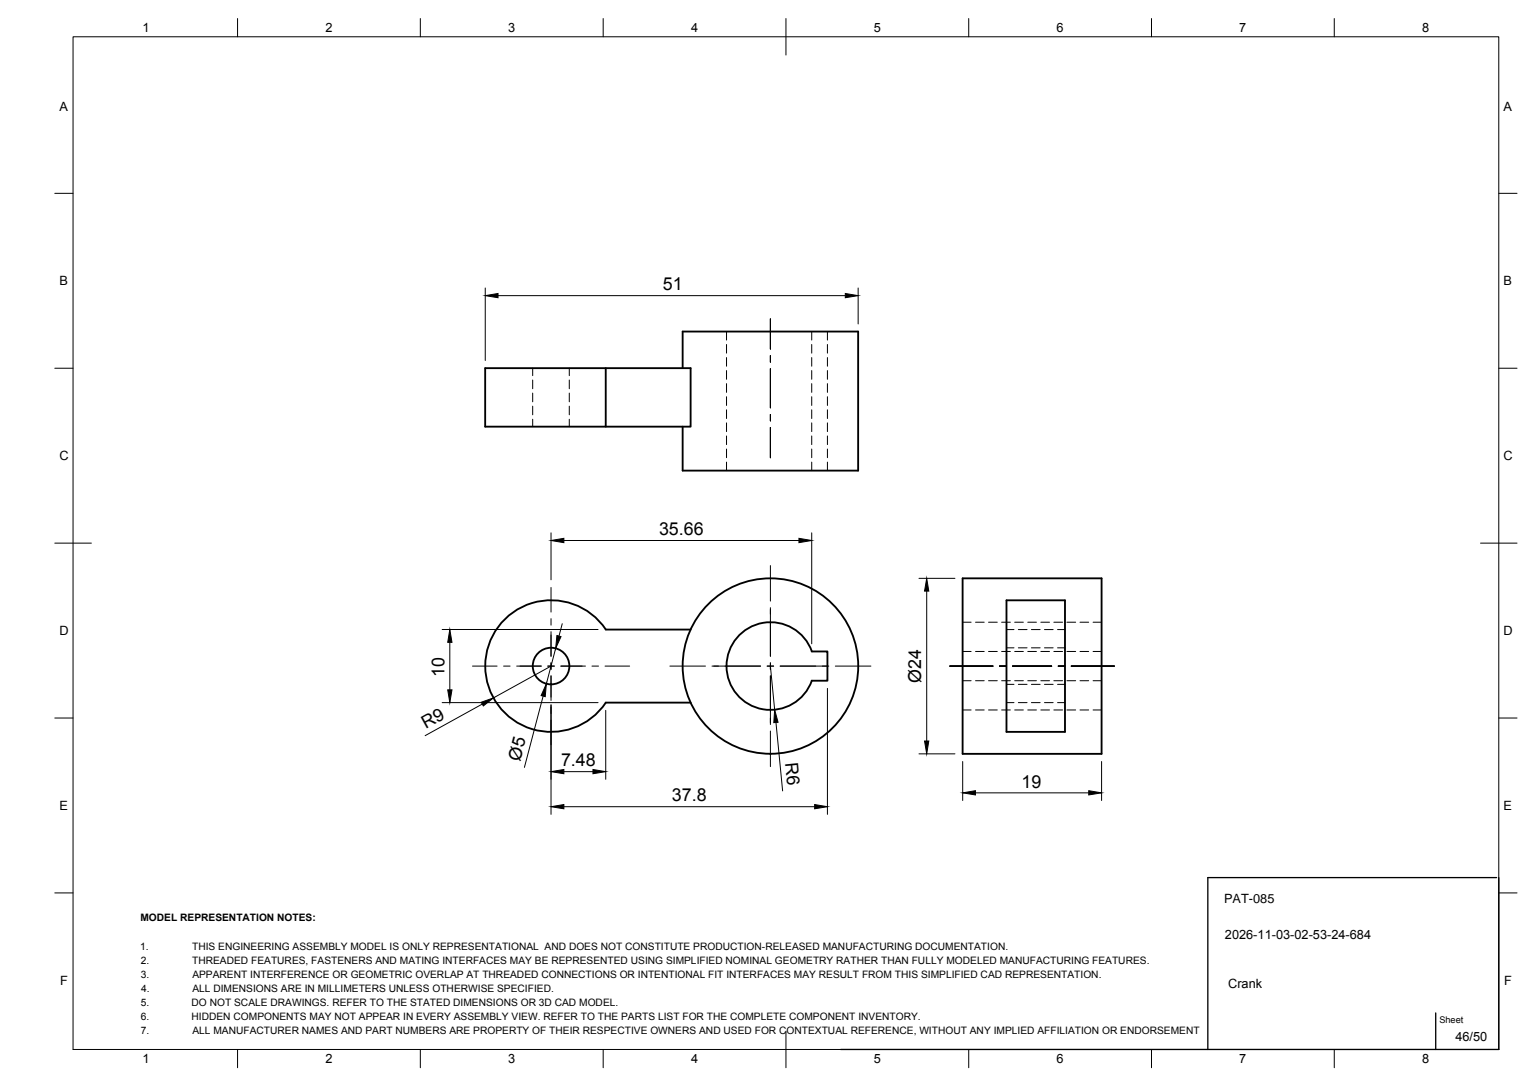
ISO-10303-21;
HEADER;
/* Generated by software containing ST-Developer
 * from STEP Tools, Inc. (www.steptools.com) 
 */

FILE_DESCRIPTION(
/* description */ ('Rack and pinion manual slide'),
/* implementation_level */ '2;1');

FILE_NAME(
/* name */ 'Crank.step',
/* time_stamp */ '2026-10-28T03:22:49-07:00',
/* author */ (''),
/* organization */ (''),
/* preprocessor_version */ 'ST-DEVELOPER v20.2',
/* originating_system */ 'Autodesk Translation Framework v15.17.0.0',
/* authorisation */ '');

FILE_SCHEMA (('AUTOMOTIVE_DESIGN { 1 0 10303 214 3 1 1 }'));
ENDSEC;

DATA;
#10=MECHANICAL_DESIGN_GEOMETRIC_PRESENTATION_REPRESENTATION('',(#777),#34851);
#678=SHAPE_REPRESENTATION_RELATIONSHIP('SRR','None',#35117,#724);
#724=ADVANCED_BREP_SHAPE_REPRESENTATION('',(#827),#34842);
#777=STYLED_ITEM('',(#35425),#827);
#827=MANIFOLD_SOLID_BREP('Body1',#13800);
#1028=FACE_BOUND('',#3056,.T.);
#1029=FACE_BOUND('',#3061,.T.);
#1030=FACE_BOUND('',#3064,.T.);
#1031=FACE_BOUND('',#3066,.T.);
#1032=FACE_BOUND('',#3068,.T.);
#1462=PLANE('',#15293);
#1463=PLANE('',#15294);
#1464=PLANE('',#15295);
#1465=PLANE('',#15296);
#1466=PLANE('',#15304);
#1467=PLANE('',#15305);
#1468=PLANE('',#15307);
#1469=PLANE('',#15308);
#1470=PLANE('',#15312);
#2117=FACE_OUTER_BOUND('',#3051,.T.);
#2118=FACE_OUTER_BOUND('',#3052,.T.);
#2119=FACE_OUTER_BOUND('',#3053,.T.);
#2120=FACE_OUTER_BOUND('',#3054,.T.);
#2121=FACE_OUTER_BOUND('',#3055,.T.);
#2122=FACE_OUTER_BOUND('',#3057,.T.);
#2123=FACE_OUTER_BOUND('',#3058,.T.);
#2124=FACE_OUTER_BOUND('',#3059,.T.);
#2125=FACE_OUTER_BOUND('',#3060,.T.);
#2126=FACE_OUTER_BOUND('',#3062,.T.);
#2127=FACE_OUTER_BOUND('',#3063,.T.);
#2128=FACE_OUTER_BOUND('',#3065,.T.);
#2129=FACE_OUTER_BOUND('',#3067,.T.);
#3051=EDGE_LOOP('',(#12062,#12063,#12064,#12065));
#3052=EDGE_LOOP('',(#12066,#12067,#12068,#12069));
#3053=EDGE_LOOP('',(#12070,#12071,#12072,#12073));
#3054=EDGE_LOOP('',(#12074,#12075,#12076,#12077));
#3055=EDGE_LOOP('',(#12078));
#3056=EDGE_LOOP('',(#12079,#12080,#12081,#12082));
#3057=EDGE_LOOP('',(#12083,#12084,#12085,#12086));
#3058=EDGE_LOOP('',(#12087,#12088,#12089,#12090));
#3059=EDGE_LOOP('',(#12091,#12092,#12093,#12094));
#3060=EDGE_LOOP('',(#12095,#12096,#12097,#12098));
#3061=EDGE_LOOP('',(#12099));
#3062=EDGE_LOOP('',(#12100,#12101,#12102,#12103));
#3063=EDGE_LOOP('',(#12104,#12105,#12106,#12107));
#3064=EDGE_LOOP('',(#12108));
#3065=EDGE_LOOP('',(#12109,#12110,#12111,#12112));
#3066=EDGE_LOOP('',(#12113,#12114,#12115,#12116));
#3067=EDGE_LOOP('',(#12117));
#3068=EDGE_LOOP('',(#12118,#12119,#12120,#12121));
#4286=LINE('',#22751,#5577);
#4287=LINE('',#22756,#5578);
#4288=LINE('',#22758,#5579);
#4289=LINE('',#22760,#5580);
#4290=LINE('',#22761,#5581);
#4291=LINE('',#22764,#5582);
#4292=LINE('',#22766,#5583);
#4293=LINE('',#22767,#5584);
#4294=LINE('',#22770,#5585);
#4295=LINE('',#22772,#5586);
#4296=LINE('',#22773,#5587);
#4297=LINE('',#22783,#5588);
#4298=LINE('',#22787,#5589);
#4299=LINE('',#22791,#5590);
#4300=LINE('',#22793,#5591);
#4301=LINE('',#22794,#5592);
#4302=LINE('',#22797,#5593);
#4303=LINE('',#22801,#5594);
#4304=LINE('',#22802,#5595);
#4305=LINE('',#22807,#5596);
#5577=VECTOR('',#18612,0.25);
#5578=VECTOR('',#18617,1.);
#5579=VECTOR('',#18618,1.);
#5580=VECTOR('',#18619,1.);
#5581=VECTOR('',#18620,1.);
#5582=VECTOR('',#18623,1.);
#5583=VECTOR('',#18624,1.);
#5584=VECTOR('',#18625,1.);
#5585=VECTOR('',#18628,1.);
#5586=VECTOR('',#18629,1.);
#5587=VECTOR('',#18630,1.);
#5588=VECTOR('',#18643,1.);
#5589=VECTOR('',#18646,1.);
#5590=VECTOR('',#18651,1.);
#5591=VECTOR('',#18652,1.);
#5592=VECTOR('',#18653,1.);
#5593=VECTOR('',#18656,1.);
#5594=VECTOR('',#18661,1.);
#5595=VECTOR('',#18662,1.);
#5596=VECTOR('',#18669,1.2);
#6142=CIRCLE('',#15291,0.25);
#6143=CIRCLE('',#15292,0.25);
#6144=CIRCLE('',#15297,1.2);
#6145=CIRCLE('',#15298,0.6);
#6146=CIRCLE('',#15300,0.6);
#6147=CIRCLE('',#15302,0.9);
#6148=CIRCLE('',#15303,0.9);
#6149=CIRCLE('',#15306,1.2);
#6150=CIRCLE('',#15309,1.2);
#6151=CIRCLE('',#15311,1.2);
#7171=VERTEX_POINT('',#22748);
#7172=VERTEX_POINT('',#22750);
#7173=VERTEX_POINT('',#22754);
#7174=VERTEX_POINT('',#22755);
#7175=VERTEX_POINT('',#22757);
#7176=VERTEX_POINT('',#22759);
#7177=VERTEX_POINT('',#22763);
#7178=VERTEX_POINT('',#22765);
#7179=VERTEX_POINT('',#22769);
#7180=VERTEX_POINT('',#22771);
#7181=VERTEX_POINT('',#22775);
#7182=VERTEX_POINT('',#22781);
#7183=VERTEX_POINT('',#22782);
#7184=VERTEX_POINT('',#22784);
#7185=VERTEX_POINT('',#22786);
#7186=VERTEX_POINT('',#22790);
#7187=VERTEX_POINT('',#22792);
#7188=VERTEX_POINT('',#22796);
#7189=VERTEX_POINT('',#22800);
#7190=VERTEX_POINT('',#22806);
#8843=EDGE_CURVE('',#7171,#7171,#6142,.T.);
#8844=EDGE_CURVE('',#7171,#7172,#4286,.T.);
#8845=EDGE_CURVE('',#7172,#7172,#6143,.T.);
#8846=EDGE_CURVE('',#7173,#7174,#4287,.T.);
#8847=EDGE_CURVE('',#7173,#7175,#4288,.T.);
#8848=EDGE_CURVE('',#7176,#7175,#4289,.T.);
#8849=EDGE_CURVE('',#7174,#7176,#4290,.T.);
#8850=EDGE_CURVE('',#7177,#7173,#4291,.T.);
#8851=EDGE_CURVE('',#7177,#7178,#4292,.T.);
#8852=EDGE_CURVE('',#7175,#7178,#4293,.T.);
#8853=EDGE_CURVE('',#7179,#7177,#4294,.T.);
#8854=EDGE_CURVE('',#7180,#7179,#4295,.T.);
#8855=EDGE_CURVE('',#7178,#7180,#4296,.T.);
#8856=EDGE_CURVE('',#7181,#7181,#6144,.T.);
#8857=EDGE_CURVE('',#7180,#7176,#6145,.T.);
#8858=EDGE_CURVE('',#7179,#7174,#6146,.T.);
#8859=EDGE_CURVE('',#7182,#7183,#4297,.T.);
#8860=EDGE_CURVE('',#7184,#7182,#6147,.T.);
#8861=EDGE_CURVE('',#7185,#7184,#4298,.T.);
#8862=EDGE_CURVE('',#7185,#7183,#6148,.T.);
#8863=EDGE_CURVE('',#7186,#7183,#4299,.T.);
#8864=EDGE_CURVE('',#7187,#7186,#4300,.T.);
#8865=EDGE_CURVE('',#7182,#7187,#4301,.T.);
#8866=EDGE_CURVE('',#7185,#7188,#4302,.T.);
#8867=EDGE_CURVE('',#7186,#7188,#6149,.T.);
#8868=EDGE_CURVE('',#7189,#7184,#4303,.T.);
#8869=EDGE_CURVE('',#7188,#7189,#4304,.T.);
#8870=EDGE_CURVE('',#7189,#7187,#6150,.T.);
#8871=EDGE_CURVE('',#7181,#7190,#4305,.T.);
#8872=EDGE_CURVE('',#7190,#7190,#6151,.T.);
#12062=ORIENTED_EDGE('',*,*,#8843,.F.);
#12063=ORIENTED_EDGE('',*,*,#8844,.T.);
#12064=ORIENTED_EDGE('',*,*,#8845,.F.);
#12065=ORIENTED_EDGE('',*,*,#8844,.F.);
#12066=ORIENTED_EDGE('',*,*,#8846,.F.);
#12067=ORIENTED_EDGE('',*,*,#8847,.T.);
#12068=ORIENTED_EDGE('',*,*,#8848,.F.);
#12069=ORIENTED_EDGE('',*,*,#8849,.F.);
#12070=ORIENTED_EDGE('',*,*,#8850,.F.);
#12071=ORIENTED_EDGE('',*,*,#8851,.T.);
#12072=ORIENTED_EDGE('',*,*,#8852,.F.);
#12073=ORIENTED_EDGE('',*,*,#8847,.F.);
#12074=ORIENTED_EDGE('',*,*,#8853,.F.);
#12075=ORIENTED_EDGE('',*,*,#8854,.F.);
#12076=ORIENTED_EDGE('',*,*,#8855,.F.);
#12077=ORIENTED_EDGE('',*,*,#8851,.F.);
#12078=ORIENTED_EDGE('',*,*,#8856,.T.);
#12079=ORIENTED_EDGE('',*,*,#8848,.T.);
#12080=ORIENTED_EDGE('',*,*,#8852,.T.);
#12081=ORIENTED_EDGE('',*,*,#8855,.T.);
#12082=ORIENTED_EDGE('',*,*,#8857,.T.);
#12083=ORIENTED_EDGE('',*,*,#8849,.T.);
#12084=ORIENTED_EDGE('',*,*,#8857,.F.);
#12085=ORIENTED_EDGE('',*,*,#8854,.T.);
#12086=ORIENTED_EDGE('',*,*,#8858,.T.);
#12087=ORIENTED_EDGE('',*,*,#8859,.F.);
#12088=ORIENTED_EDGE('',*,*,#8860,.F.);
#12089=ORIENTED_EDGE('',*,*,#8861,.F.);
#12090=ORIENTED_EDGE('',*,*,#8862,.T.);
#12091=ORIENTED_EDGE('',*,*,#8859,.T.);
#12092=ORIENTED_EDGE('',*,*,#8863,.F.);
#12093=ORIENTED_EDGE('',*,*,#8864,.F.);
#12094=ORIENTED_EDGE('',*,*,#8865,.F.);
#12095=ORIENTED_EDGE('',*,*,#8862,.F.);
#12096=ORIENTED_EDGE('',*,*,#8866,.T.);
#12097=ORIENTED_EDGE('',*,*,#8867,.F.);
#12098=ORIENTED_EDGE('',*,*,#8863,.T.);
#12099=ORIENTED_EDGE('',*,*,#8843,.T.);
#12100=ORIENTED_EDGE('',*,*,#8861,.T.);
#12101=ORIENTED_EDGE('',*,*,#8868,.F.);
#12102=ORIENTED_EDGE('',*,*,#8869,.F.);
#12103=ORIENTED_EDGE('',*,*,#8866,.F.);
#12104=ORIENTED_EDGE('',*,*,#8865,.T.);
#12105=ORIENTED_EDGE('',*,*,#8870,.F.);
#12106=ORIENTED_EDGE('',*,*,#8868,.T.);
#12107=ORIENTED_EDGE('',*,*,#8860,.T.);
#12108=ORIENTED_EDGE('',*,*,#8845,.T.);
#12109=ORIENTED_EDGE('',*,*,#8856,.F.);
#12110=ORIENTED_EDGE('',*,*,#8871,.T.);
#12111=ORIENTED_EDGE('',*,*,#8872,.T.);
#12112=ORIENTED_EDGE('',*,*,#8871,.F.);
#12113=ORIENTED_EDGE('',*,*,#8864,.T.);
#12114=ORIENTED_EDGE('',*,*,#8867,.T.);
#12115=ORIENTED_EDGE('',*,*,#8869,.T.);
#12116=ORIENTED_EDGE('',*,*,#8870,.T.);
#12117=ORIENTED_EDGE('',*,*,#8872,.F.);
#12118=ORIENTED_EDGE('',*,*,#8846,.T.);
#12119=ORIENTED_EDGE('',*,*,#8858,.F.);
#12120=ORIENTED_EDGE('',*,*,#8853,.T.);
#12121=ORIENTED_EDGE('',*,*,#8850,.T.);
#12977=CYLINDRICAL_SURFACE('',#15290,0.25);
#12978=CYLINDRICAL_SURFACE('',#15299,0.6);
#12979=CYLINDRICAL_SURFACE('',#15301,0.9);
#12980=CYLINDRICAL_SURFACE('',#15310,1.2);
#13595=ADVANCED_FACE('',(#2117),#12977,.F.);
#13596=ADVANCED_FACE('',(#2118),#1462,.F.);
#13597=ADVANCED_FACE('',(#2119),#1463,.F.);
#13598=ADVANCED_FACE('',(#2120),#1464,.F.);
#13599=ADVANCED_FACE('',(#2121,#1028),#1465,.T.);
#13600=ADVANCED_FACE('',(#2122),#12978,.F.);
#13601=ADVANCED_FACE('',(#2123),#12979,.T.);
#13602=ADVANCED_FACE('',(#2124),#1466,.T.);
#13603=ADVANCED_FACE('',(#2125,#1029),#1467,.F.);
#13604=ADVANCED_FACE('',(#2126),#1468,.T.);
#13605=ADVANCED_FACE('',(#2127,#1030),#1469,.T.);
#13606=ADVANCED_FACE('',(#2128,#1031),#12980,.T.);
#13607=ADVANCED_FACE('',(#2129,#1032),#1470,.F.);
#13800=CLOSED_SHELL('',(#13595,#13596,#13597,#13598,#13599,#13600,#13601,
#13602,#13603,#13604,#13605,#13606,#13607));
#15289=AXIS2_PLACEMENT_3D('',#22746,#18606,#18607);
#15290=AXIS2_PLACEMENT_3D('',#22747,#18608,#18609);
#15291=AXIS2_PLACEMENT_3D('',#22749,#18610,#18611);
#15292=AXIS2_PLACEMENT_3D('',#22752,#18613,#18614);
#15293=AXIS2_PLACEMENT_3D('',#22753,#18615,#18616);
#15294=AXIS2_PLACEMENT_3D('',#22762,#18621,#18622);
#15295=AXIS2_PLACEMENT_3D('',#22768,#18626,#18627);
#15296=AXIS2_PLACEMENT_3D('',#22774,#18631,#18632);
#15297=AXIS2_PLACEMENT_3D('',#22776,#18633,#18634);
#15298=AXIS2_PLACEMENT_3D('',#22777,#18635,#18636);
#15299=AXIS2_PLACEMENT_3D('',#22778,#18637,#18638);
#15300=AXIS2_PLACEMENT_3D('',#22779,#18639,#18640);
#15301=AXIS2_PLACEMENT_3D('',#22780,#18641,#18642);
#15302=AXIS2_PLACEMENT_3D('',#22785,#18644,#18645);
#15303=AXIS2_PLACEMENT_3D('',#22788,#18647,#18648);
#15304=AXIS2_PLACEMENT_3D('',#22789,#18649,#18650);
#15305=AXIS2_PLACEMENT_3D('',#22795,#18654,#18655);
#15306=AXIS2_PLACEMENT_3D('',#22798,#18657,#18658);
#15307=AXIS2_PLACEMENT_3D('',#22799,#18659,#18660);
#15308=AXIS2_PLACEMENT_3D('',#22803,#18663,#18664);
#15309=AXIS2_PLACEMENT_3D('',#22804,#18665,#18666);
#15310=AXIS2_PLACEMENT_3D('',#22805,#18667,#18668);
#15311=AXIS2_PLACEMENT_3D('',#22808,#18670,#18671);
#15312=AXIS2_PLACEMENT_3D('',#22809,#18672,#18673);
#18606=DIRECTION('axis',(0.,0.,1.));
#18607=DIRECTION('refdir',(1.,0.,0.));
#18608=DIRECTION('center_axis',(0.,1.,0.));
#18609=DIRECTION('ref_axis',(1.,0.,0.));
#18610=DIRECTION('center_axis',(0.,1.,0.));
#18611=DIRECTION('ref_axis',(1.,0.,0.));
#18612=DIRECTION('',(0.,1.,0.));
#18613=DIRECTION('center_axis',(0.,-1.,0.));
#18614=DIRECTION('ref_axis',(1.,0.,0.));
#18615=DIRECTION('center_axis',(-1.,0.,0.));
#18616=DIRECTION('ref_axis',(0.,0.,1.));
#18617=DIRECTION('',(0.,0.,1.));
#18618=DIRECTION('',(0.,1.,0.));
#18619=DIRECTION('',(0.,0.,-1.));
#18620=DIRECTION('',(0.,1.,0.));
#18621=DIRECTION('center_axis',(0.,0.,-1.));
#18622=DIRECTION('ref_axis',(-1.,0.,0.));
#18623=DIRECTION('',(-1.,0.,0.));
#18624=DIRECTION('',(0.,1.,0.));
#18625=DIRECTION('',(1.,0.,0.));
#18626=DIRECTION('center_axis',(1.,0.,0.));
#18627=DIRECTION('ref_axis',(0.,0.,-1.));
#18628=DIRECTION('',(0.,0.,-1.));
#18629=DIRECTION('',(0.,-1.,0.));
#18630=DIRECTION('',(0.,0.,1.));
#18631=DIRECTION('center_axis',(0.,1.,0.));
#18632=DIRECTION('ref_axis',(1.,0.,0.));
#18633=DIRECTION('center_axis',(0.,1.,0.));
#18634=DIRECTION('ref_axis',(1.,0.,0.));
#18635=DIRECTION('center_axis',(0.,-1.,0.));
#18636=DIRECTION('ref_axis',(1.,0.,0.));
#18637=DIRECTION('center_axis',(0.,1.,0.));
#18638=DIRECTION('ref_axis',(-1.83697019872103E-16,0.,1.));
#18639=DIRECTION('center_axis',(0.,-1.,0.));
#18640=DIRECTION('ref_axis',(1.,0.,0.));
#18641=DIRECTION('center_axis',(0.,1.,0.));
#18642=DIRECTION('ref_axis',(6.12323399573677E-17,0.,1.));
#18643=DIRECTION('',(0.,-1.,0.));
#18644=DIRECTION('center_axis',(0.,1.,0.));
#18645=DIRECTION('ref_axis',(1.,0.,0.));
#18646=DIRECTION('',(0.,1.,0.));
#18647=DIRECTION('center_axis',(0.,1.,0.));
#18648=DIRECTION('ref_axis',(1.,0.,0.));
#18649=DIRECTION('center_axis',(1.,0.,0.));
#18650=DIRECTION('ref_axis',(0.,0.,-1.));
#18651=DIRECTION('',(0.,0.,1.));
#18652=DIRECTION('',(0.,-1.,0.));
#18653=DIRECTION('',(0.,0.,-1.));
#18654=DIRECTION('center_axis',(0.,1.,0.));
#18655=DIRECTION('ref_axis',(1.,0.,0.));
#18656=DIRECTION('',(0.,0.,-1.));
#18657=DIRECTION('center_axis',(0.,-1.,0.));
#18658=DIRECTION('ref_axis',(1.,0.,0.));
#18659=DIRECTION('center_axis',(-1.,0.,0.));
#18660=DIRECTION('ref_axis',(0.,0.,1.));
#18661=DIRECTION('',(0.,0.,1.));
#18662=DIRECTION('',(0.,1.,0.));
#18663=DIRECTION('center_axis',(0.,1.,0.));
#18664=DIRECTION('ref_axis',(0.,0.,1.));
#18665=DIRECTION('center_axis',(0.,1.,0.));
#18666=DIRECTION('ref_axis',(1.,0.,0.));
#18667=DIRECTION('center_axis',(0.,1.,0.));
#18668=DIRECTION('ref_axis',(1.,0.,0.));
#18669=DIRECTION('',(0.,-1.,0.));
#18670=DIRECTION('center_axis',(0.,1.,0.));
#18671=DIRECTION('ref_axis',(1.,0.,0.));
#18672=DIRECTION('center_axis',(0.,1.,0.));
#18673=DIRECTION('ref_axis',(1.,0.,0.));
#22746=CARTESIAN_POINT('',(0.,0.,0.));
#22747=CARTESIAN_POINT('Origin',(11.,6.4,13.25));
#22748=CARTESIAN_POINT('',(10.75,6.5,13.25));
#22749=CARTESIAN_POINT('Origin',(11.,6.5,13.25));
#22750=CARTESIAN_POINT('',(10.75,7.3,13.25));
#22751=CARTESIAN_POINT('',(10.75,6.4,13.25));
#22752=CARTESIAN_POINT('Origin',(11.,7.3,13.25));
#22753=CARTESIAN_POINT('Origin',(10.8,5.9,9.47));
#22754=CARTESIAN_POINT('',(10.8,6.,9.47));
#22755=CARTESIAN_POINT('',(10.8,6.,9.68431457505076));
#22756=CARTESIAN_POINT('',(10.8,6.,9.86));
#22757=CARTESIAN_POINT('',(10.8,7.9,9.47));
#22758=CARTESIAN_POINT('',(10.8,5.9,9.47));
#22759=CARTESIAN_POINT('',(10.8,7.9,9.68431457505076));
#22760=CARTESIAN_POINT('',(10.8,7.9,9.86));
#22761=CARTESIAN_POINT('',(10.8,6.,9.68431457505076));
#22762=CARTESIAN_POINT('Origin',(11.2,5.9,9.47));
#22763=CARTESIAN_POINT('',(11.2,6.,9.47));
#22764=CARTESIAN_POINT('',(11.1,6.,9.47));
#22765=CARTESIAN_POINT('',(11.2,7.9,9.47));
#22766=CARTESIAN_POINT('',(11.2,5.9,9.47));
#22767=CARTESIAN_POINT('',(11.1,7.9,9.47));
#22768=CARTESIAN_POINT('Origin',(11.2,5.9,10.25));
#22769=CARTESIAN_POINT('',(11.2,6.,9.68431457505076));
#22770=CARTESIAN_POINT('',(11.2,6.,10.25));
#22771=CARTESIAN_POINT('',(11.2,7.9,9.68431457505076));
#22772=CARTESIAN_POINT('',(11.2,6.,9.68431457505076));
#22773=CARTESIAN_POINT('',(11.2,7.9,10.25));
#22774=CARTESIAN_POINT('Origin',(11.,7.9,10.25));
#22775=CARTESIAN_POINT('',(9.8,7.9,10.25));
#22776=CARTESIAN_POINT('Origin',(11.,7.9,10.25));
#22777=CARTESIAN_POINT('Origin',(11.,7.9,10.25));
#22778=CARTESIAN_POINT('Origin',(11.,6.,10.25));
#22779=CARTESIAN_POINT('Origin',(11.,6.,10.25));
#22780=CARTESIAN_POINT('Origin',(11.,6.5,13.25));
#22781=CARTESIAN_POINT('',(11.5,7.3,12.5016685226452));
#22782=CARTESIAN_POINT('',(11.5,6.5,12.5016685226452));
#22783=CARTESIAN_POINT('',(11.5,6.5,12.5016685226452));
#22784=CARTESIAN_POINT('',(10.5,7.3,12.5016685226452));
#22785=CARTESIAN_POINT('Origin',(11.,7.3,13.25));
#22786=CARTESIAN_POINT('',(10.5,6.5,12.5016685226452));
#22787=CARTESIAN_POINT('',(10.5,6.5,12.5016685226452));
#22788=CARTESIAN_POINT('Origin',(11.,6.5,13.25));
#22789=CARTESIAN_POINT('Origin',(11.5,6.5,13.25));
#22790=CARTESIAN_POINT('',(11.5,6.5,11.3408712114636));
#22791=CARTESIAN_POINT('',(11.5,6.5,10.25));
#22792=CARTESIAN_POINT('',(11.5,7.3,11.3408712114636));
#22793=CARTESIAN_POINT('',(11.5,6.,11.3408712114636));
#22794=CARTESIAN_POINT('',(11.5,7.3,10.25));
#22795=CARTESIAN_POINT('Origin',(11.,6.5,11.75));
#22796=CARTESIAN_POINT('',(10.5,6.5,11.3408712114636));
#22797=CARTESIAN_POINT('',(10.5,6.5,13.25));
#22798=CARTESIAN_POINT('Origin',(11.,6.5,10.25));
#22799=CARTESIAN_POINT('Origin',(10.5,6.5,10.25));
#22800=CARTESIAN_POINT('',(10.5,7.3,11.3408712114636));
#22801=CARTESIAN_POINT('',(10.5,7.3,13.25));
#22802=CARTESIAN_POINT('',(10.5,6.,11.3408712114636));
#22803=CARTESIAN_POINT('Origin',(11.,7.3,11.75));
#22804=CARTESIAN_POINT('Origin',(11.,7.3,10.25));
#22805=CARTESIAN_POINT('Origin',(11.,6.,10.25));
#22806=CARTESIAN_POINT('',(9.8,6.,10.25));
#22807=CARTESIAN_POINT('',(9.8,6.,10.25));
#22808=CARTESIAN_POINT('Origin',(11.,6.,10.25));
#22809=CARTESIAN_POINT('Origin',(11.,6.,10.25));
#34788=UNCERTAINTY_MEASURE_WITH_UNIT(LENGTH_MEASURE(0.001),#34852,
'DISTANCE_ACCURACY_VALUE',
'Maximum model space distance between geometric entities at asserted c
onnectivities');
#34797=UNCERTAINTY_MEASURE_WITH_UNIT(LENGTH_MEASURE(0.001),#34852,
'DISTANCE_ACCURACY_VALUE',
'Maximum model space distance between geometric entities at asserted c
onnectivities');
#34842=(
GEOMETRIC_REPRESENTATION_CONTEXT(3)
GLOBAL_UNCERTAINTY_ASSIGNED_CONTEXT((#34788))
GLOBAL_UNIT_ASSIGNED_CONTEXT((#34852,#34854,#34855))
REPRESENTATION_CONTEXT('','3D')
);
#34851=(
GEOMETRIC_REPRESENTATION_CONTEXT(3)
GLOBAL_UNCERTAINTY_ASSIGNED_CONTEXT((#34797))
GLOBAL_UNIT_ASSIGNED_CONTEXT((#34852,#34854,#34855))
REPRESENTATION_CONTEXT('','3D')
);
#34852=(
LENGTH_UNIT()
NAMED_UNIT(*)
SI_UNIT(.CENTI.,.METRE.)
);
#34854=(
NAMED_UNIT(*)
PLANE_ANGLE_UNIT()
SI_UNIT($,.RADIAN.)
);
#34855=(
NAMED_UNIT(*)
SI_UNIT($,.STERADIAN.)
SOLID_ANGLE_UNIT()
);
#34900=SHAPE_DEFINITION_REPRESENTATION(#34961,#35117);
#34961=PRODUCT_DEFINITION_SHAPE('',$,#35171);
#35117=SHAPE_REPRESENTATION('',(#15289),#34842);
#35126=PRODUCT_DEFINITION_CONTEXT('part definition',#35287,'design');
#35171=PRODUCT_DEFINITION('Crank','Crank',#35224,#35126);
#35224=PRODUCT_DEFINITION_FORMATION('',$,#35333);
#35287=APPLICATION_CONTEXT(
'Core Data for Automotive Mechanical Design Process');
#35288=PRODUCT_CONTEXT('part definition',#35287,'mechanical');
#35333=PRODUCT('Crank','Crank','Crank',(#35288));
#35419=COLOUR_RGB('Off White',0.89,0.88,0.83);
#35420=FILL_AREA_STYLE_COLOUR('',#35419);
#35421=FILL_AREA_STYLE('',(#35420));
#35422=SURFACE_STYLE_FILL_AREA(#35421);
#35423=SURFACE_SIDE_STYLE('',(#35422));
#35424=SURFACE_STYLE_USAGE(.BOTH.,#35423);
#35425=PRESENTATION_STYLE_ASSIGNMENT((#35424));
ENDSEC;
END-ISO-10303-21;
